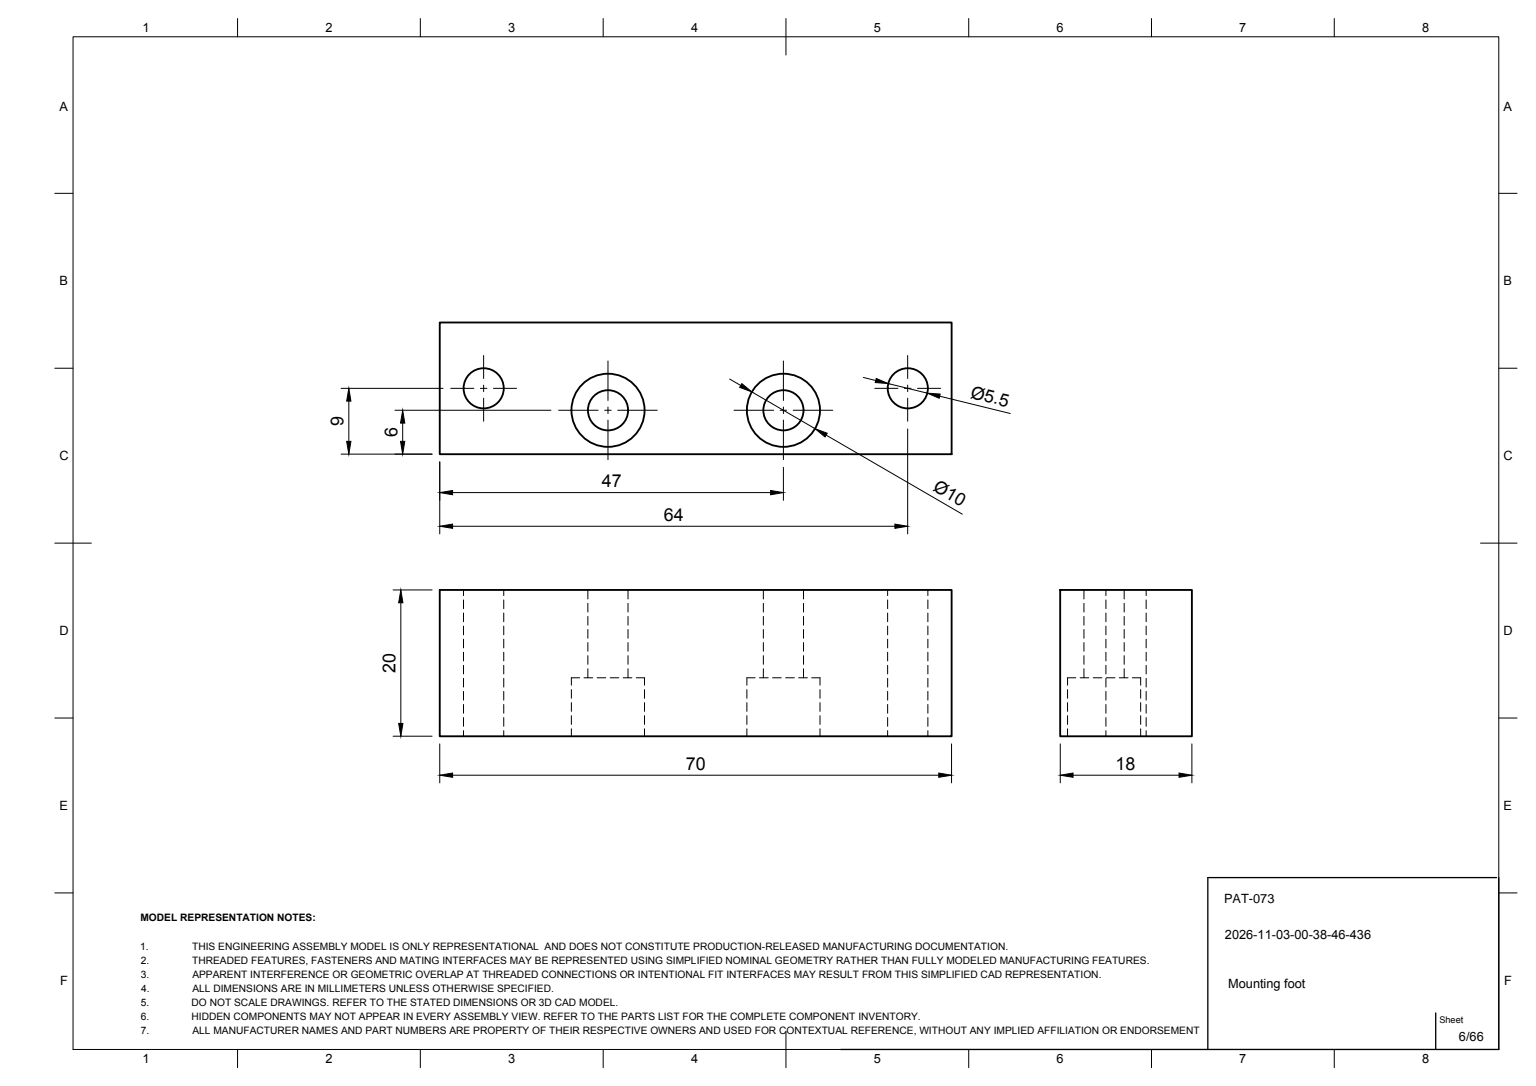
ISO-10303-21;
HEADER;
/* Generated by software containing ST-Developer
 * from STEP Tools, Inc. (www.steptools.com) 
 */

FILE_DESCRIPTION(
/* description */ ('Manual piston pump'),
/* implementation_level */ '2;1');

FILE_NAME(
/* name */ 'Mounting foot.step',
/* time_stamp */ '2026-11-02T16:54:23-08:00',
/* author */ (''),
/* organization */ (''),
/* preprocessor_version */ 'ST-DEVELOPER v20.2',
/* originating_system */ 'Autodesk Translation Framework v15.17.0.0',
/* authorisation */ '');

FILE_SCHEMA (('AUTOMOTIVE_DESIGN { 1 0 10303 214 3 1 1 }'));
ENDSEC;

DATA;
#10=MECHANICAL_DESIGN_GEOMETRIC_PRESENTATION_REPRESENTATION('',(#689),#19043);
#563=SHAPE_REPRESENTATION_RELATIONSHIP('SRR','None',#19309,#626);
#626=ADVANCED_BREP_SHAPE_REPRESENTATION('',(#761),#18976);
#689=STYLED_ITEM('',(#19662),#761);
#761=MANIFOLD_SOLID_BREP('Body1',#9473);
#840=FACE_BOUND('',#1908,.T.);
#841=FACE_BOUND('',#1911,.T.);
#842=FACE_BOUND('',#1919,.T.);
#843=FACE_BOUND('',#1920,.T.);
#844=FACE_BOUND('',#1921,.T.);
#845=FACE_BOUND('',#1922,.T.);
#846=FACE_BOUND('',#1924,.T.);
#847=FACE_BOUND('',#1925,.T.);
#848=FACE_BOUND('',#1926,.T.);
#849=FACE_BOUND('',#1927,.T.);
#1103=CYLINDRICAL_SURFACE('',#10296,0.275);
#1104=CYLINDRICAL_SURFACE('',#10299,0.275);
#1105=CYLINDRICAL_SURFACE('',#10302,0.5);
#1106=CYLINDRICAL_SURFACE('',#10307,0.5);
#1107=CYLINDRICAL_SURFACE('',#10312,0.275);
#1108=CYLINDRICAL_SURFACE('',#10314,0.275);
#1316=FACE_OUTER_BOUND('',#1904,.T.);
#1317=FACE_OUTER_BOUND('',#1905,.T.);
#1318=FACE_OUTER_BOUND('',#1906,.T.);
#1319=FACE_OUTER_BOUND('',#1907,.T.);
#1320=FACE_OUTER_BOUND('',#1909,.T.);
#1321=FACE_OUTER_BOUND('',#1910,.T.);
#1322=FACE_OUTER_BOUND('',#1912,.T.);
#1323=FACE_OUTER_BOUND('',#1913,.T.);
#1324=FACE_OUTER_BOUND('',#1914,.T.);
#1325=FACE_OUTER_BOUND('',#1915,.T.);
#1326=FACE_OUTER_BOUND('',#1916,.T.);
#1327=FACE_OUTER_BOUND('',#1917,.T.);
#1328=FACE_OUTER_BOUND('',#1918,.T.);
#1329=FACE_OUTER_BOUND('',#1923,.T.);
#1904=EDGE_LOOP('',(#6397,#6398,#6399,#6400));
#1905=EDGE_LOOP('',(#6401,#6402,#6403,#6404));
#1906=EDGE_LOOP('',(#6405,#6406,#6407,#6408));
#1907=EDGE_LOOP('',(#6409));
#1908=EDGE_LOOP('',(#6410));
#1909=EDGE_LOOP('',(#6411,#6412,#6413,#6414));
#1910=EDGE_LOOP('',(#6415));
#1911=EDGE_LOOP('',(#6416));
#1912=EDGE_LOOP('',(#6417,#6418,#6419,#6420));
#1913=EDGE_LOOP('',(#6421,#6422,#6423,#6424));
#1914=EDGE_LOOP('',(#6425,#6426,#6427,#6428));
#1915=EDGE_LOOP('',(#6429,#6430,#6431,#6432));
#1916=EDGE_LOOP('',(#6433,#6434,#6435,#6436));
#1917=EDGE_LOOP('',(#6437,#6438,#6439,#6440));
#1918=EDGE_LOOP('',(#6441,#6442,#6443,#6444));
#1919=EDGE_LOOP('',(#6445));
#1920=EDGE_LOOP('',(#6446));
#1921=EDGE_LOOP('',(#6447));
#1922=EDGE_LOOP('',(#6448));
#1923=EDGE_LOOP('',(#6449,#6450,#6451,#6452));
#1924=EDGE_LOOP('',(#6453));
#1925=EDGE_LOOP('',(#6454));
#1926=EDGE_LOOP('',(#6455));
#1927=EDGE_LOOP('',(#6456));
#2688=CIRCLE('',#10297,0.275);
#2689=CIRCLE('',#10298,0.275);
#2690=CIRCLE('',#10300,0.275);
#2691=CIRCLE('',#10301,0.275);
#2692=CIRCLE('',#10303,0.5);
#2693=CIRCLE('',#10304,0.5);
#2694=CIRCLE('',#10306,0.275);
#2695=CIRCLE('',#10308,0.5);
#2696=CIRCLE('',#10309,0.5);
#2697=CIRCLE('',#10311,0.275);
#2698=CIRCLE('',#10313,0.275);
#2699=CIRCLE('',#10315,0.275);
#3182=LINE('',#14772,#3786);
#3183=LINE('',#14778,#3787);
#3184=LINE('',#14784,#3788);
#3185=LINE('',#14793,#3789);
#3186=LINE('',#14800,#3790);
#3187=LINE('',#14804,#3791);
#3188=LINE('',#14809,#3792);
#3189=LINE('',#14811,#3793);
#3190=LINE('',#14813,#3794);
#3191=LINE('',#14814,#3795);
#3192=LINE('',#14817,#3796);
#3193=LINE('',#14819,#3797);
#3194=LINE('',#14820,#3798);
#3195=LINE('',#14823,#3799);
#3196=LINE('',#14825,#3800);
#3197=LINE('',#14826,#3801);
#3198=LINE('',#14828,#3802);
#3199=LINE('',#14829,#3803);
#3786=VECTOR('',#11640,0.275);
#3787=VECTOR('',#11647,0.275);
#3788=VECTOR('',#11654,0.5);
#3789=VECTOR('',#11665,0.5);
#3790=VECTOR('',#11674,0.275);
#3791=VECTOR('',#11679,0.275);
#3792=VECTOR('',#11684,1.);
#3793=VECTOR('',#11685,1.);
#3794=VECTOR('',#11686,1.);
#3795=VECTOR('',#11687,1.);
#3796=VECTOR('',#11690,1.);
#3797=VECTOR('',#11691,1.);
#3798=VECTOR('',#11692,1.);
#3799=VECTOR('',#11695,1.);
#3800=VECTOR('',#11696,1.);
#3801=VECTOR('',#11697,1.);
#3802=VECTOR('',#11700,1.);
#3803=VECTOR('',#11701,1.);
#4396=VERTEX_POINT('',#14769);
#4397=VERTEX_POINT('',#14771);
#4398=VERTEX_POINT('',#14775);
#4399=VERTEX_POINT('',#14777);
#4400=VERTEX_POINT('',#14781);
#4401=VERTEX_POINT('',#14783);
#4402=VERTEX_POINT('',#14787);
#4403=VERTEX_POINT('',#14790);
#4404=VERTEX_POINT('',#14792);
#4405=VERTEX_POINT('',#14796);
#4406=VERTEX_POINT('',#14799);
#4407=VERTEX_POINT('',#14803);
#4408=VERTEX_POINT('',#14807);
#4409=VERTEX_POINT('',#14808);
#4410=VERTEX_POINT('',#14810);
#4411=VERTEX_POINT('',#14812);
#4412=VERTEX_POINT('',#14816);
#4413=VERTEX_POINT('',#14818);
#4414=VERTEX_POINT('',#14822);
#4415=VERTEX_POINT('',#14824);
#5185=EDGE_CURVE('',#4396,#4396,#2688,.T.);
#5186=EDGE_CURVE('',#4396,#4397,#3182,.T.);
#5187=EDGE_CURVE('',#4397,#4397,#2689,.T.);
#5188=EDGE_CURVE('',#4398,#4398,#2690,.T.);
#5189=EDGE_CURVE('',#4398,#4399,#3183,.T.);
#5190=EDGE_CURVE('',#4399,#4399,#2691,.T.);
#5191=EDGE_CURVE('',#4400,#4400,#2692,.T.);
#5192=EDGE_CURVE('',#4400,#4401,#3184,.T.);
#5193=EDGE_CURVE('',#4401,#4401,#2693,.T.);
#5194=EDGE_CURVE('',#4402,#4402,#2694,.T.);
#5195=EDGE_CURVE('',#4403,#4403,#2695,.T.);
#5196=EDGE_CURVE('',#4403,#4404,#3185,.T.);
#5197=EDGE_CURVE('',#4404,#4404,#2696,.T.);
#5198=EDGE_CURVE('',#4405,#4405,#2697,.T.);
#5199=EDGE_CURVE('',#4402,#4406,#3186,.T.);
#5200=EDGE_CURVE('',#4406,#4406,#2698,.T.);
#5201=EDGE_CURVE('',#4405,#4407,#3187,.T.);
#5202=EDGE_CURVE('',#4407,#4407,#2699,.T.);
#5203=EDGE_CURVE('',#4408,#4409,#3188,.T.);
#5204=EDGE_CURVE('',#4409,#4410,#3189,.T.);
#5205=EDGE_CURVE('',#4411,#4410,#3190,.T.);
#5206=EDGE_CURVE('',#4408,#4411,#3191,.T.);
#5207=EDGE_CURVE('',#4412,#4408,#3192,.T.);
#5208=EDGE_CURVE('',#4413,#4411,#3193,.T.);
#5209=EDGE_CURVE('',#4412,#4413,#3194,.T.);
#5210=EDGE_CURVE('',#4414,#4412,#3195,.T.);
#5211=EDGE_CURVE('',#4415,#4413,#3196,.T.);
#5212=EDGE_CURVE('',#4414,#4415,#3197,.T.);
#5213=EDGE_CURVE('',#4409,#4414,#3198,.T.);
#5214=EDGE_CURVE('',#4410,#4415,#3199,.T.);
#6397=ORIENTED_EDGE('',*,*,#5185,.F.);
#6398=ORIENTED_EDGE('',*,*,#5186,.T.);
#6399=ORIENTED_EDGE('',*,*,#5187,.F.);
#6400=ORIENTED_EDGE('',*,*,#5186,.F.);
#6401=ORIENTED_EDGE('',*,*,#5188,.F.);
#6402=ORIENTED_EDGE('',*,*,#5189,.T.);
#6403=ORIENTED_EDGE('',*,*,#5190,.F.);
#6404=ORIENTED_EDGE('',*,*,#5189,.F.);
#6405=ORIENTED_EDGE('',*,*,#5191,.F.);
#6406=ORIENTED_EDGE('',*,*,#5192,.T.);
#6407=ORIENTED_EDGE('',*,*,#5193,.T.);
#6408=ORIENTED_EDGE('',*,*,#5192,.F.);
#6409=ORIENTED_EDGE('',*,*,#5193,.F.);
#6410=ORIENTED_EDGE('',*,*,#5194,.F.);
#6411=ORIENTED_EDGE('',*,*,#5195,.F.);
#6412=ORIENTED_EDGE('',*,*,#5196,.T.);
#6413=ORIENTED_EDGE('',*,*,#5197,.T.);
#6414=ORIENTED_EDGE('',*,*,#5196,.F.);
#6415=ORIENTED_EDGE('',*,*,#5197,.F.);
#6416=ORIENTED_EDGE('',*,*,#5198,.F.);
#6417=ORIENTED_EDGE('',*,*,#5194,.T.);
#6418=ORIENTED_EDGE('',*,*,#5199,.T.);
#6419=ORIENTED_EDGE('',*,*,#5200,.F.);
#6420=ORIENTED_EDGE('',*,*,#5199,.F.);
#6421=ORIENTED_EDGE('',*,*,#5198,.T.);
#6422=ORIENTED_EDGE('',*,*,#5201,.T.);
#6423=ORIENTED_EDGE('',*,*,#5202,.F.);
#6424=ORIENTED_EDGE('',*,*,#5201,.F.);
#6425=ORIENTED_EDGE('',*,*,#5203,.T.);
#6426=ORIENTED_EDGE('',*,*,#5204,.T.);
#6427=ORIENTED_EDGE('',*,*,#5205,.F.);
#6428=ORIENTED_EDGE('',*,*,#5206,.F.);
#6429=ORIENTED_EDGE('',*,*,#5207,.T.);
#6430=ORIENTED_EDGE('',*,*,#5206,.T.);
#6431=ORIENTED_EDGE('',*,*,#5208,.F.);
#6432=ORIENTED_EDGE('',*,*,#5209,.F.);
#6433=ORIENTED_EDGE('',*,*,#5210,.T.);
#6434=ORIENTED_EDGE('',*,*,#5209,.T.);
#6435=ORIENTED_EDGE('',*,*,#5211,.F.);
#6436=ORIENTED_EDGE('',*,*,#5212,.F.);
#6437=ORIENTED_EDGE('',*,*,#5213,.T.);
#6438=ORIENTED_EDGE('',*,*,#5212,.T.);
#6439=ORIENTED_EDGE('',*,*,#5214,.F.);
#6440=ORIENTED_EDGE('',*,*,#5204,.F.);
#6441=ORIENTED_EDGE('',*,*,#5214,.T.);
#6442=ORIENTED_EDGE('',*,*,#5211,.T.);
#6443=ORIENTED_EDGE('',*,*,#5208,.T.);
#6444=ORIENTED_EDGE('',*,*,#5205,.T.);
#6445=ORIENTED_EDGE('',*,*,#5187,.T.);
#6446=ORIENTED_EDGE('',*,*,#5190,.T.);
#6447=ORIENTED_EDGE('',*,*,#5200,.T.);
#6448=ORIENTED_EDGE('',*,*,#5202,.T.);
#6449=ORIENTED_EDGE('',*,*,#5213,.F.);
#6450=ORIENTED_EDGE('',*,*,#5203,.F.);
#6451=ORIENTED_EDGE('',*,*,#5207,.F.);
#6452=ORIENTED_EDGE('',*,*,#5210,.F.);
#6453=ORIENTED_EDGE('',*,*,#5185,.T.);
#6454=ORIENTED_EDGE('',*,*,#5188,.T.);
#6455=ORIENTED_EDGE('',*,*,#5191,.T.);
#6456=ORIENTED_EDGE('',*,*,#5195,.T.);
#8585=PLANE('',#10305);
#8586=PLANE('',#10310);
#8587=PLANE('',#10316);
#8588=PLANE('',#10317);
#8589=PLANE('',#10318);
#8590=PLANE('',#10319);
#8591=PLANE('',#10320);
#8592=PLANE('',#10321);
#8921=ADVANCED_FACE('',(#1316),#1103,.F.);
#8922=ADVANCED_FACE('',(#1317),#1104,.F.);
#8923=ADVANCED_FACE('',(#1318),#1105,.F.);
#8924=ADVANCED_FACE('',(#1319,#840),#8585,.F.);
#8925=ADVANCED_FACE('',(#1320),#1106,.F.);
#8926=ADVANCED_FACE('',(#1321,#841),#8586,.F.);
#8927=ADVANCED_FACE('',(#1322),#1107,.F.);
#8928=ADVANCED_FACE('',(#1323),#1108,.F.);
#8929=ADVANCED_FACE('',(#1324),#8587,.T.);
#8930=ADVANCED_FACE('',(#1325),#8588,.T.);
#8931=ADVANCED_FACE('',(#1326),#8589,.T.);
#8932=ADVANCED_FACE('',(#1327),#8590,.T.);
#8933=ADVANCED_FACE('',(#1328,#842,#843,#844,#845),#8591,.T.);
#8934=ADVANCED_FACE('',(#1329,#846,#847,#848,#849),#8592,.F.);
#9473=CLOSED_SHELL('',(#8921,#8922,#8923,#8924,#8925,#8926,#8927,#8928,
#8929,#8930,#8931,#8932,#8933,#8934));
#10295=AXIS2_PLACEMENT_3D('',#14767,#11634,#11635);
#10296=AXIS2_PLACEMENT_3D('',#14768,#11636,#11637);
#10297=AXIS2_PLACEMENT_3D('',#14770,#11638,#11639);
#10298=AXIS2_PLACEMENT_3D('',#14773,#11641,#11642);
#10299=AXIS2_PLACEMENT_3D('',#14774,#11643,#11644);
#10300=AXIS2_PLACEMENT_3D('',#14776,#11645,#11646);
#10301=AXIS2_PLACEMENT_3D('',#14779,#11648,#11649);
#10302=AXIS2_PLACEMENT_3D('',#14780,#11650,#11651);
#10303=AXIS2_PLACEMENT_3D('',#14782,#11652,#11653);
#10304=AXIS2_PLACEMENT_3D('',#14785,#11655,#11656);
#10305=AXIS2_PLACEMENT_3D('',#14786,#11657,#11658);
#10306=AXIS2_PLACEMENT_3D('',#14788,#11659,#11660);
#10307=AXIS2_PLACEMENT_3D('',#14789,#11661,#11662);
#10308=AXIS2_PLACEMENT_3D('',#14791,#11663,#11664);
#10309=AXIS2_PLACEMENT_3D('',#14794,#11666,#11667);
#10310=AXIS2_PLACEMENT_3D('',#14795,#11668,#11669);
#10311=AXIS2_PLACEMENT_3D('',#14797,#11670,#11671);
#10312=AXIS2_PLACEMENT_3D('',#14798,#11672,#11673);
#10313=AXIS2_PLACEMENT_3D('',#14801,#11675,#11676);
#10314=AXIS2_PLACEMENT_3D('',#14802,#11677,#11678);
#10315=AXIS2_PLACEMENT_3D('',#14805,#11680,#11681);
#10316=AXIS2_PLACEMENT_3D('',#14806,#11682,#11683);
#10317=AXIS2_PLACEMENT_3D('',#14815,#11688,#11689);
#10318=AXIS2_PLACEMENT_3D('',#14821,#11693,#11694);
#10319=AXIS2_PLACEMENT_3D('',#14827,#11698,#11699);
#10320=AXIS2_PLACEMENT_3D('',#14830,#11702,#11703);
#10321=AXIS2_PLACEMENT_3D('',#14831,#11704,#11705);
#11634=DIRECTION('axis',(0.,0.,1.));
#11635=DIRECTION('refdir',(1.,0.,0.));
#11636=DIRECTION('center_axis',(0.,0.,1.));
#11637=DIRECTION('ref_axis',(1.,0.,0.));
#11638=DIRECTION('center_axis',(0.,0.,1.));
#11639=DIRECTION('ref_axis',(1.,0.,0.));
#11640=DIRECTION('',(0.,0.,1.));
#11641=DIRECTION('center_axis',(0.,0.,-1.));
#11642=DIRECTION('ref_axis',(1.,0.,0.));
#11643=DIRECTION('center_axis',(0.,0.,1.));
#11644=DIRECTION('ref_axis',(1.,0.,0.));
#11645=DIRECTION('center_axis',(0.,0.,1.));
#11646=DIRECTION('ref_axis',(1.,0.,0.));
#11647=DIRECTION('',(0.,0.,1.));
#11648=DIRECTION('center_axis',(0.,0.,-1.));
#11649=DIRECTION('ref_axis',(1.,0.,0.));
#11650=DIRECTION('center_axis',(0.,0.,1.));
#11651=DIRECTION('ref_axis',(1.,0.,0.));
#11652=DIRECTION('center_axis',(0.,0.,1.));
#11653=DIRECTION('ref_axis',(1.,0.,0.));
#11654=DIRECTION('',(0.,0.,1.));
#11655=DIRECTION('center_axis',(0.,0.,1.));
#11656=DIRECTION('ref_axis',(1.,0.,0.));
#11657=DIRECTION('center_axis',(0.,0.,1.));
#11658=DIRECTION('ref_axis',(1.,0.,0.));
#11659=DIRECTION('center_axis',(0.,0.,-1.));
#11660=DIRECTION('ref_axis',(1.,0.,0.));
#11661=DIRECTION('center_axis',(0.,0.,1.));
#11662=DIRECTION('ref_axis',(1.,0.,0.));
#11663=DIRECTION('center_axis',(0.,0.,1.));
#11664=DIRECTION('ref_axis',(1.,0.,0.));
#11665=DIRECTION('',(0.,0.,1.));
#11666=DIRECTION('center_axis',(0.,0.,1.));
#11667=DIRECTION('ref_axis',(1.,0.,0.));
#11668=DIRECTION('center_axis',(0.,0.,1.));
#11669=DIRECTION('ref_axis',(1.,0.,0.));
#11670=DIRECTION('center_axis',(0.,0.,-1.));
#11671=DIRECTION('ref_axis',(1.,0.,0.));
#11672=DIRECTION('center_axis',(0.,0.,1.));
#11673=DIRECTION('ref_axis',(1.,0.,0.));
#11674=DIRECTION('',(0.,0.,1.));
#11675=DIRECTION('center_axis',(0.,0.,-1.));
#11676=DIRECTION('ref_axis',(1.,0.,0.));
#11677=DIRECTION('center_axis',(0.,0.,1.));
#11678=DIRECTION('ref_axis',(1.,0.,0.));
#11679=DIRECTION('',(0.,0.,1.));
#11680=DIRECTION('center_axis',(0.,0.,-1.));
#11681=DIRECTION('ref_axis',(1.,0.,0.));
#11682=DIRECTION('center_axis',(0.,1.,0.));
#11683=DIRECTION('ref_axis',(-1.,0.,0.));
#11684=DIRECTION('',(-1.,0.,0.));
#11685=DIRECTION('',(0.,0.,1.));
#11686=DIRECTION('',(-1.,0.,0.));
#11687=DIRECTION('',(0.,0.,1.));
#11688=DIRECTION('center_axis',(1.,0.,0.));
#11689=DIRECTION('ref_axis',(0.,1.,0.));
#11690=DIRECTION('',(0.,1.,0.));
#11691=DIRECTION('',(0.,1.,0.));
#11692=DIRECTION('',(0.,0.,1.));
#11693=DIRECTION('center_axis',(0.,-1.,0.));
#11694=DIRECTION('ref_axis',(1.,0.,0.));
#11695=DIRECTION('',(1.,0.,0.));
#11696=DIRECTION('',(1.,0.,0.));
#11697=DIRECTION('',(0.,0.,1.));
#11698=DIRECTION('center_axis',(-1.,0.,0.));
#11699=DIRECTION('ref_axis',(0.,-1.,0.));
#11700=DIRECTION('',(0.,-1.,0.));
#11701=DIRECTION('',(0.,-1.,0.));
#11702=DIRECTION('center_axis',(0.,0.,1.));
#11703=DIRECTION('ref_axis',(1.,0.,0.));
#11704=DIRECTION('center_axis',(0.,0.,1.));
#11705=DIRECTION('ref_axis',(1.,0.,0.));
#14767=CARTESIAN_POINT('',(0.,0.,0.));
#14768=CARTESIAN_POINT('Origin',(-2.9,0.9,-0.1));
#14769=CARTESIAN_POINT('',(-3.175,0.9,0.));
#14770=CARTESIAN_POINT('Origin',(-2.9,0.9,0.));
#14771=CARTESIAN_POINT('',(-3.175,0.9,2.));
#14772=CARTESIAN_POINT('',(-3.175,0.9,-0.1));
#14773=CARTESIAN_POINT('Origin',(-2.9,0.9,2.));
#14774=CARTESIAN_POINT('Origin',(2.9,0.9,-0.1));
#14775=CARTESIAN_POINT('',(2.625,0.9,0.));
#14776=CARTESIAN_POINT('Origin',(2.9,0.9,0.));
#14777=CARTESIAN_POINT('',(2.625,0.9,2.));
#14778=CARTESIAN_POINT('',(2.625,0.9,-0.1));
#14779=CARTESIAN_POINT('Origin',(2.9,0.9,2.));
#14780=CARTESIAN_POINT('Origin',(-1.2,0.6,-0.1));
#14781=CARTESIAN_POINT('',(-1.7,0.6,0.));
#14782=CARTESIAN_POINT('Origin',(-1.2,0.6,0.));
#14783=CARTESIAN_POINT('',(-1.7,0.6,0.8));
#14784=CARTESIAN_POINT('',(-1.7,0.6,-0.1));
#14785=CARTESIAN_POINT('Origin',(-1.2,0.6,0.8));
#14786=CARTESIAN_POINT('Origin',(-1.2,0.6,0.8));
#14787=CARTESIAN_POINT('',(-1.475,0.6,0.8));
#14788=CARTESIAN_POINT('Origin',(-1.2,0.6,0.8));
#14789=CARTESIAN_POINT('Origin',(1.2,0.6,-0.1));
#14790=CARTESIAN_POINT('',(0.7,0.6,0.));
#14791=CARTESIAN_POINT('Origin',(1.2,0.6,0.));
#14792=CARTESIAN_POINT('',(0.7,0.6,0.8));
#14793=CARTESIAN_POINT('',(0.7,0.6,-0.1));
#14794=CARTESIAN_POINT('Origin',(1.2,0.6,0.8));
#14795=CARTESIAN_POINT('Origin',(1.2,0.6,0.8));
#14796=CARTESIAN_POINT('',(0.925,0.6,0.8));
#14797=CARTESIAN_POINT('Origin',(1.2,0.6,0.8));
#14798=CARTESIAN_POINT('Origin',(-1.2,0.6,-0.1));
#14799=CARTESIAN_POINT('',(-1.475,0.6,2.));
#14800=CARTESIAN_POINT('',(-1.475,0.6,-0.1));
#14801=CARTESIAN_POINT('Origin',(-1.2,0.6,2.));
#14802=CARTESIAN_POINT('Origin',(1.2,0.6,-0.1));
#14803=CARTESIAN_POINT('',(0.925,0.6,2.));
#14804=CARTESIAN_POINT('',(0.925,0.6,-0.1));
#14805=CARTESIAN_POINT('Origin',(1.2,0.6,2.));
#14806=CARTESIAN_POINT('Origin',(3.5,1.8,0.));
#14807=CARTESIAN_POINT('',(3.5,1.8,0.));
#14808=CARTESIAN_POINT('',(-3.5,1.8,0.));
#14809=CARTESIAN_POINT('',(3.5,1.8,0.));
#14810=CARTESIAN_POINT('',(-3.5,1.8,2.));
#14811=CARTESIAN_POINT('',(-3.5,1.8,0.));
#14812=CARTESIAN_POINT('',(3.5,1.8,2.));
#14813=CARTESIAN_POINT('',(3.5,1.8,2.));
#14814=CARTESIAN_POINT('',(3.5,1.8,0.));
#14815=CARTESIAN_POINT('Origin',(3.5,0.,0.));
#14816=CARTESIAN_POINT('',(3.5,0.,0.));
#14817=CARTESIAN_POINT('',(3.5,0.,0.));
#14818=CARTESIAN_POINT('',(3.5,0.,2.));
#14819=CARTESIAN_POINT('',(3.5,0.,2.));
#14820=CARTESIAN_POINT('',(3.5,0.,0.));
#14821=CARTESIAN_POINT('Origin',(-3.5,0.,0.));
#14822=CARTESIAN_POINT('',(-3.5,0.,0.));
#14823=CARTESIAN_POINT('',(-3.5,0.,0.));
#14824=CARTESIAN_POINT('',(-3.5,0.,2.));
#14825=CARTESIAN_POINT('',(-3.5,0.,2.));
#14826=CARTESIAN_POINT('',(-3.5,0.,0.));
#14827=CARTESIAN_POINT('Origin',(-3.5,1.8,0.));
#14828=CARTESIAN_POINT('',(-3.5,1.8,0.));
#14829=CARTESIAN_POINT('',(-3.5,1.8,2.));
#14830=CARTESIAN_POINT('Origin',(0.,0.9,2.));
#14831=CARTESIAN_POINT('Origin',(0.,0.9,0.));
#18905=UNCERTAINTY_MEASURE_WITH_UNIT(LENGTH_MEASURE(0.001),#19044,
'DISTANCE_ACCURACY_VALUE',
'Maximum model space distance between geometric entities at asserted c
onnectivities');
#18972=UNCERTAINTY_MEASURE_WITH_UNIT(LENGTH_MEASURE(0.001),#19044,
'DISTANCE_ACCURACY_VALUE',
'Maximum model space distance between geometric entities at asserted c
onnectivities');
#18976=(
GEOMETRIC_REPRESENTATION_CONTEXT(3)
GLOBAL_UNCERTAINTY_ASSIGNED_CONTEXT((#18905))
GLOBAL_UNIT_ASSIGNED_CONTEXT((#19044,#19046,#19047))
REPRESENTATION_CONTEXT('','3D')
);
#19043=(
GEOMETRIC_REPRESENTATION_CONTEXT(3)
GLOBAL_UNCERTAINTY_ASSIGNED_CONTEXT((#18972))
GLOBAL_UNIT_ASSIGNED_CONTEXT((#19044,#19046,#19047))
REPRESENTATION_CONTEXT('','3D')
);
#19044=(
LENGTH_UNIT()
NAMED_UNIT(*)
SI_UNIT(.CENTI.,.METRE.)
);
#19046=(
NAMED_UNIT(*)
PLANE_ANGLE_UNIT()
SI_UNIT($,.RADIAN.)
);
#19047=(
NAMED_UNIT(*)
SI_UNIT($,.STERADIAN.)
SOLID_ANGLE_UNIT()
);
#19051=SHAPE_DEFINITION_REPRESENTATION(#19121,#19309);
#19121=PRODUCT_DEFINITION_SHAPE('',$,#19380);
#19309=SHAPE_REPRESENTATION('',(#10295),#18976);
#19376=PRODUCT_DEFINITION_CONTEXT('part definition',#19588,'design');
#19380=PRODUCT_DEFINITION('2026-11-03-00-38-46-436','Mounting foot',#19450,
#19376);
#19450=PRODUCT_DEFINITION_FORMATION('',$,#19593);
#19588=APPLICATION_CONTEXT(
'Core Data for Automotive Mechanical Design Process');
#19589=PRODUCT_CONTEXT('part definition',#19588,'mechanical');
#19593=PRODUCT('2026-11-03-00-38-46-436','Mounting foot',
'Mounting foot',(#19589));
#19662=PRESENTATION_STYLE_ASSIGNMENT((#19668));
#19668=SURFACE_STYLE_USAGE(.BOTH.,#19674);
#19674=SURFACE_SIDE_STYLE('',(#19680));
#19680=SURFACE_STYLE_FILL_AREA(#19686);
#19686=FILL_AREA_STYLE('CAD Library Painted - Deep blue',(#19692));
#19692=FILL_AREA_STYLE_COLOUR('CAD Library Painted - Deep blue',#19698);
#19698=COLOUR_RGB('CAD Library Painted - Deep blue',0.0784313725490196,
0.203921568627451,0.349019607843137);
ENDSEC;
END-ISO-10303-21;
